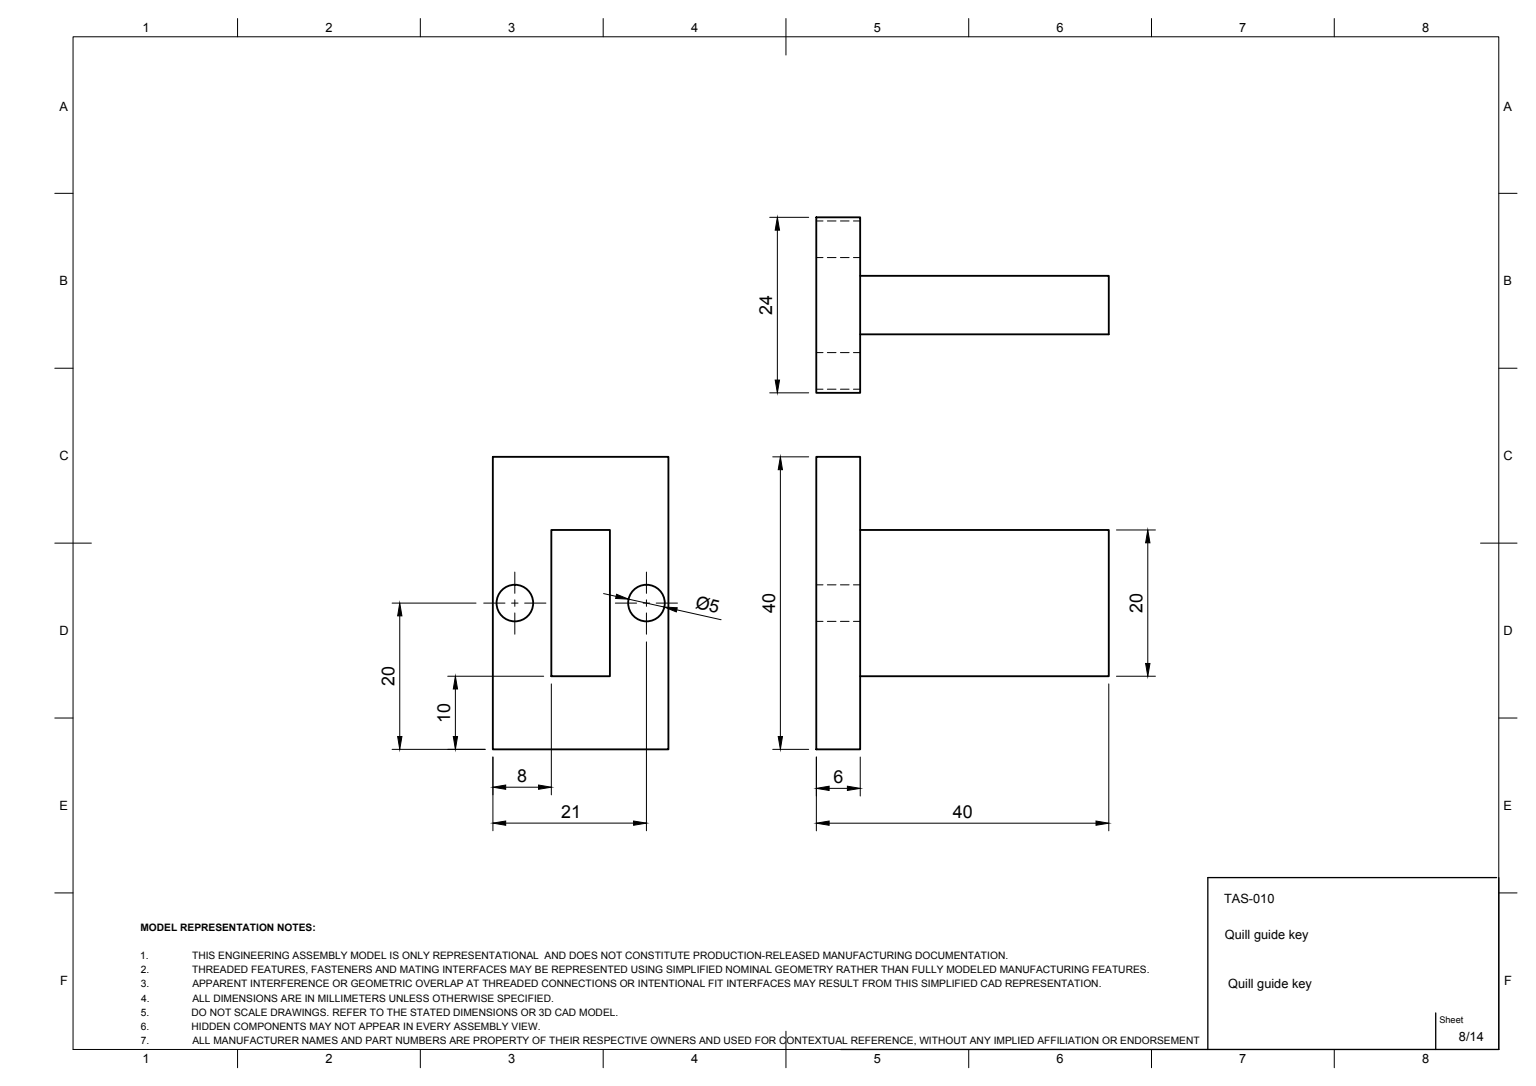
ISO-10303-21;
HEADER;
/* Generated by software containing ST-Developer
 * from STEP Tools, Inc. (www.steptools.com) 
 */

FILE_DESCRIPTION(
/* description */ (
'Independent keyed-quill tailstock, native coupled50mm slider andM16x2
 feed screw, conical dead center, bronze sleeves/thrust washers, cross
-pinned handwheel and bolted guide key. Custom center taper; no standa
rd taper compatibility, machine-bed compatibility or load rating assig
ned.'),
/* implementation_level */ '2;1');

FILE_NAME(
/* name */ 'Quill guide key.step',
/* time_stamp */ '2026-11-14T07:17:36-08:00',
/* author */ (''),
/* organization */ (''),
/* preprocessor_version */ 'ST-DEVELOPER v20.2',
/* originating_system */ 'Autodesk Translation Framework v15.17.0.0',
/* authorisation */ '');

FILE_SCHEMA (('AUTOMOTIVE_DESIGN { 1 0 10303 214 3 1 1 }'));
ENDSEC;

DATA;
#10=MECHANICAL_DESIGN_GEOMETRIC_PRESENTATION_REPRESENTATION('',(#158),#289387);
#124=SHAPE_REPRESENTATION_RELATIONSHIP('SRR','None',#289459,#141);
#141=ADVANCED_BREP_SHAPE_REPRESENTATION('',(#175),#289375);
#158=STYLED_ITEM('',(#289552),#175);
#175=MANIFOLD_SOLID_BREP('Body1',#16846);
#223=FACE_BOUND('',#1527,.T.);
#224=FACE_BOUND('',#1528,.T.);
#225=FACE_BOUND('',#1529,.T.);
#226=FACE_BOUND('',#1535,.T.);
#227=FACE_BOUND('',#1536,.T.);
#354=PLANE('',#17542);
#355=PLANE('',#17543);
#356=PLANE('',#17544);
#357=PLANE('',#17545);
#358=PLANE('',#17546);
#359=PLANE('',#17547);
#360=PLANE('',#17548);
#361=PLANE('',#17549);
#362=PLANE('',#17550);
#363=PLANE('',#17551);
#364=PLANE('',#17552);
#838=FACE_OUTER_BOUND('',#1524,.T.);
#839=FACE_OUTER_BOUND('',#1525,.T.);
#840=FACE_OUTER_BOUND('',#1526,.T.);
#841=FACE_OUTER_BOUND('',#1530,.T.);
#842=FACE_OUTER_BOUND('',#1531,.T.);
#843=FACE_OUTER_BOUND('',#1532,.T.);
#844=FACE_OUTER_BOUND('',#1533,.T.);
#845=FACE_OUTER_BOUND('',#1534,.T.);
#846=FACE_OUTER_BOUND('',#1537,.T.);
#847=FACE_OUTER_BOUND('',#1538,.T.);
#848=FACE_OUTER_BOUND('',#1539,.T.);
#849=FACE_OUTER_BOUND('',#1540,.T.);
#850=FACE_OUTER_BOUND('',#1541,.T.);
#1524=EDGE_LOOP('',(#13673,#13674,#13675,#13676));
#1525=EDGE_LOOP('',(#13677,#13678,#13679,#13680));
#1526=EDGE_LOOP('',(#13681,#13682,#13683,#13684));
#1527=EDGE_LOOP('',(#13685));
#1528=EDGE_LOOP('',(#13686));
#1529=EDGE_LOOP('',(#13687,#13688,#13689,#13690));
#1530=EDGE_LOOP('',(#13691,#13692,#13693,#13694));
#1531=EDGE_LOOP('',(#13695,#13696,#13697,#13698));
#1532=EDGE_LOOP('',(#13699,#13700,#13701,#13702));
#1533=EDGE_LOOP('',(#13703,#13704,#13705,#13706));
#1534=EDGE_LOOP('',(#13707,#13708,#13709,#13710));
#1535=EDGE_LOOP('',(#13711));
#1536=EDGE_LOOP('',(#13712));
#1537=EDGE_LOOP('',(#13713,#13714,#13715,#13716));
#1538=EDGE_LOOP('',(#13717,#13718,#13719,#13720));
#1539=EDGE_LOOP('',(#13721,#13722,#13723,#13724));
#1540=EDGE_LOOP('',(#13725,#13726,#13727,#13728));
#1541=EDGE_LOOP('',(#13729,#13730,#13731,#13732));
#1899=CIRCLE('',#17537,2.5);
#1900=CIRCLE('',#17538,2.5);
#1901=CIRCLE('',#17540,2.5);
#1902=CIRCLE('',#17541,2.5);
#4329=LINE('',#185169,#4966);
#4330=LINE('',#185175,#4967);
#4331=LINE('',#185180,#4968);
#4332=LINE('',#185182,#4969);
#4333=LINE('',#185184,#4970);
#4334=LINE('',#185185,#4971);
#4335=LINE('',#185188,#4972);
#4336=LINE('',#185190,#4973);
#4337=LINE('',#185192,#4974);
#4338=LINE('',#185193,#4975);
#4339=LINE('',#185196,#4976);
#4340=LINE('',#185198,#4977);
#4341=LINE('',#185199,#4978);
#4342=LINE('',#185202,#4979);
#4343=LINE('',#185203,#4980);
#4344=LINE('',#185206,#4981);
#4345=LINE('',#185207,#4982);
#4346=LINE('',#185209,#4983);
#4347=LINE('',#185214,#4984);
#4348=LINE('',#185215,#4985);
#4349=LINE('',#185216,#4986);
#4350=LINE('',#185219,#4987);
#4351=LINE('',#185220,#4988);
#4352=LINE('',#185223,#4989);
#4353=LINE('',#185224,#4990);
#4354=LINE('',#185226,#4991);
#4966=VECTOR('',#19261,2.5);
#4967=VECTOR('',#19268,2.5);
#4968=VECTOR('',#19273,10.);
#4969=VECTOR('',#19274,10.);
#4970=VECTOR('',#19275,10.);
#4971=VECTOR('',#19276,10.);
#4972=VECTOR('',#19277,10.);
#4973=VECTOR('',#19278,10.);
#4974=VECTOR('',#19279,10.);
#4975=VECTOR('',#19280,10.);
#4976=VECTOR('',#19283,10.);
#4977=VECTOR('',#19284,10.);
#4978=VECTOR('',#19285,10.);
#4979=VECTOR('',#19288,10.);
#4980=VECTOR('',#19289,10.);
#4981=VECTOR('',#19292,10.);
#4982=VECTOR('',#19293,10.);
#4983=VECTOR('',#19296,10.);
#4984=VECTOR('',#19301,10.);
#4985=VECTOR('',#19302,10.);
#4986=VECTOR('',#19303,10.);
#4987=VECTOR('',#19306,10.);
#4988=VECTOR('',#19307,10.);
#4989=VECTOR('',#19310,10.);
#4990=VECTOR('',#19311,10.);
#4991=VECTOR('',#19314,10.);
#6580=VERTEX_POINT('',#185166);
#6581=VERTEX_POINT('',#185168);
#6582=VERTEX_POINT('',#185172);
#6583=VERTEX_POINT('',#185174);
#6584=VERTEX_POINT('',#185178);
#6585=VERTEX_POINT('',#185179);
#6586=VERTEX_POINT('',#185181);
#6587=VERTEX_POINT('',#185183);
#6588=VERTEX_POINT('',#185186);
#6589=VERTEX_POINT('',#185187);
#6590=VERTEX_POINT('',#185189);
#6591=VERTEX_POINT('',#185191);
#6592=VERTEX_POINT('',#185195);
#6593=VERTEX_POINT('',#185197);
#6594=VERTEX_POINT('',#185201);
#6595=VERTEX_POINT('',#185205);
#6596=VERTEX_POINT('',#185212);
#6597=VERTEX_POINT('',#185213);
#6598=VERTEX_POINT('',#185218);
#6599=VERTEX_POINT('',#185222);
#9148=EDGE_CURVE('',#6580,#6580,#1899,.T.);
#9149=EDGE_CURVE('',#6580,#6581,#4329,.T.);
#9150=EDGE_CURVE('',#6581,#6581,#1900,.T.);
#9151=EDGE_CURVE('',#6582,#6582,#1901,.T.);
#9152=EDGE_CURVE('',#6582,#6583,#4330,.T.);
#9153=EDGE_CURVE('',#6583,#6583,#1902,.T.);
#9154=EDGE_CURVE('',#6584,#6585,#4331,.T.);
#9155=EDGE_CURVE('',#6586,#6584,#4332,.T.);
#9156=EDGE_CURVE('',#6587,#6586,#4333,.T.);
#9157=EDGE_CURVE('',#6585,#6587,#4334,.T.);
#9158=EDGE_CURVE('',#6588,#6589,#4335,.T.);
#9159=EDGE_CURVE('',#6589,#6590,#4336,.T.);
#9160=EDGE_CURVE('',#6590,#6591,#4337,.T.);
#9161=EDGE_CURVE('',#6591,#6588,#4338,.T.);
#9162=EDGE_CURVE('',#6584,#6592,#4339,.T.);
#9163=EDGE_CURVE('',#6593,#6592,#4340,.T.);
#9164=EDGE_CURVE('',#6586,#6593,#4341,.T.);
#9165=EDGE_CURVE('',#6594,#6593,#4342,.T.);
#9166=EDGE_CURVE('',#6587,#6594,#4343,.T.);
#9167=EDGE_CURVE('',#6595,#6594,#4344,.T.);
#9168=EDGE_CURVE('',#6585,#6595,#4345,.T.);
#9169=EDGE_CURVE('',#6592,#6595,#4346,.T.);
#9170=EDGE_CURVE('',#6596,#6597,#4347,.T.);
#9171=EDGE_CURVE('',#6597,#6589,#4348,.T.);
#9172=EDGE_CURVE('',#6596,#6588,#4349,.T.);
#9173=EDGE_CURVE('',#6598,#6596,#4350,.T.);
#9174=EDGE_CURVE('',#6598,#6591,#4351,.T.);
#9175=EDGE_CURVE('',#6599,#6598,#4352,.T.);
#9176=EDGE_CURVE('',#6599,#6590,#4353,.T.);
#9177=EDGE_CURVE('',#6597,#6599,#4354,.T.);
#13673=ORIENTED_EDGE('',*,*,#9148,.F.);
#13674=ORIENTED_EDGE('',*,*,#9149,.T.);
#13675=ORIENTED_EDGE('',*,*,#9150,.F.);
#13676=ORIENTED_EDGE('',*,*,#9149,.F.);
#13677=ORIENTED_EDGE('',*,*,#9151,.F.);
#13678=ORIENTED_EDGE('',*,*,#9152,.T.);
#13679=ORIENTED_EDGE('',*,*,#9153,.F.);
#13680=ORIENTED_EDGE('',*,*,#9152,.F.);
#13681=ORIENTED_EDGE('',*,*,#9154,.F.);
#13682=ORIENTED_EDGE('',*,*,#9155,.F.);
#13683=ORIENTED_EDGE('',*,*,#9156,.F.);
#13684=ORIENTED_EDGE('',*,*,#9157,.F.);
#13685=ORIENTED_EDGE('',*,*,#9150,.T.);
#13686=ORIENTED_EDGE('',*,*,#9153,.T.);
#13687=ORIENTED_EDGE('',*,*,#9158,.T.);
#13688=ORIENTED_EDGE('',*,*,#9159,.T.);
#13689=ORIENTED_EDGE('',*,*,#9160,.T.);
#13690=ORIENTED_EDGE('',*,*,#9161,.T.);
#13691=ORIENTED_EDGE('',*,*,#9155,.T.);
#13692=ORIENTED_EDGE('',*,*,#9162,.T.);
#13693=ORIENTED_EDGE('',*,*,#9163,.F.);
#13694=ORIENTED_EDGE('',*,*,#9164,.F.);
#13695=ORIENTED_EDGE('',*,*,#9156,.T.);
#13696=ORIENTED_EDGE('',*,*,#9164,.T.);
#13697=ORIENTED_EDGE('',*,*,#9165,.F.);
#13698=ORIENTED_EDGE('',*,*,#9166,.F.);
#13699=ORIENTED_EDGE('',*,*,#9157,.T.);
#13700=ORIENTED_EDGE('',*,*,#9166,.T.);
#13701=ORIENTED_EDGE('',*,*,#9167,.F.);
#13702=ORIENTED_EDGE('',*,*,#9168,.F.);
#13703=ORIENTED_EDGE('',*,*,#9154,.T.);
#13704=ORIENTED_EDGE('',*,*,#9168,.T.);
#13705=ORIENTED_EDGE('',*,*,#9169,.F.);
#13706=ORIENTED_EDGE('',*,*,#9162,.F.);
#13707=ORIENTED_EDGE('',*,*,#9169,.T.);
#13708=ORIENTED_EDGE('',*,*,#9167,.T.);
#13709=ORIENTED_EDGE('',*,*,#9165,.T.);
#13710=ORIENTED_EDGE('',*,*,#9163,.T.);
#13711=ORIENTED_EDGE('',*,*,#9148,.T.);
#13712=ORIENTED_EDGE('',*,*,#9151,.T.);
#13713=ORIENTED_EDGE('',*,*,#9170,.T.);
#13714=ORIENTED_EDGE('',*,*,#9171,.T.);
#13715=ORIENTED_EDGE('',*,*,#9158,.F.);
#13716=ORIENTED_EDGE('',*,*,#9172,.F.);
#13717=ORIENTED_EDGE('',*,*,#9173,.T.);
#13718=ORIENTED_EDGE('',*,*,#9172,.T.);
#13719=ORIENTED_EDGE('',*,*,#9161,.F.);
#13720=ORIENTED_EDGE('',*,*,#9174,.F.);
#13721=ORIENTED_EDGE('',*,*,#9175,.T.);
#13722=ORIENTED_EDGE('',*,*,#9174,.T.);
#13723=ORIENTED_EDGE('',*,*,#9160,.F.);
#13724=ORIENTED_EDGE('',*,*,#9176,.F.);
#13725=ORIENTED_EDGE('',*,*,#9177,.T.);
#13726=ORIENTED_EDGE('',*,*,#9176,.T.);
#13727=ORIENTED_EDGE('',*,*,#9159,.F.);
#13728=ORIENTED_EDGE('',*,*,#9171,.F.);
#13729=ORIENTED_EDGE('',*,*,#9177,.F.);
#13730=ORIENTED_EDGE('',*,*,#9170,.F.);
#13731=ORIENTED_EDGE('',*,*,#9173,.F.);
#13732=ORIENTED_EDGE('',*,*,#9175,.F.);
#16038=CYLINDRICAL_SURFACE('',#17536,2.5);
#16039=CYLINDRICAL_SURFACE('',#17539,2.5);
#16606=ADVANCED_FACE('',(#838),#16038,.F.);
#16607=ADVANCED_FACE('',(#839),#16039,.F.);
#16608=ADVANCED_FACE('',(#840,#223,#224,#225),#354,.F.);
#16609=ADVANCED_FACE('',(#841),#355,.T.);
#16610=ADVANCED_FACE('',(#842),#356,.T.);
#16611=ADVANCED_FACE('',(#843),#357,.T.);
#16612=ADVANCED_FACE('',(#844),#358,.T.);
#16613=ADVANCED_FACE('',(#845,#226,#227),#359,.T.);
#16614=ADVANCED_FACE('',(#846),#360,.T.);
#16615=ADVANCED_FACE('',(#847),#361,.T.);
#16616=ADVANCED_FACE('',(#848),#362,.T.);
#16617=ADVANCED_FACE('',(#849),#363,.T.);
#16618=ADVANCED_FACE('',(#850),#364,.F.);
#16846=CLOSED_SHELL('',(#16606,#16607,#16608,#16609,#16610,#16611,#16612,
#16613,#16614,#16615,#16616,#16617,#16618));
#17535=AXIS2_PLACEMENT_3D('',#185164,#19255,#19256);
#17536=AXIS2_PLACEMENT_3D('',#185165,#19257,#19258);
#17537=AXIS2_PLACEMENT_3D('',#185167,#19259,#19260);
#17538=AXIS2_PLACEMENT_3D('',#185170,#19262,#19263);
#17539=AXIS2_PLACEMENT_3D('',#185171,#19264,#19265);
#17540=AXIS2_PLACEMENT_3D('',#185173,#19266,#19267);
#17541=AXIS2_PLACEMENT_3D('',#185176,#19269,#19270);
#17542=AXIS2_PLACEMENT_3D('',#185177,#19271,#19272);
#17543=AXIS2_PLACEMENT_3D('',#185194,#19281,#19282);
#17544=AXIS2_PLACEMENT_3D('',#185200,#19286,#19287);
#17545=AXIS2_PLACEMENT_3D('',#185204,#19290,#19291);
#17546=AXIS2_PLACEMENT_3D('',#185208,#19294,#19295);
#17547=AXIS2_PLACEMENT_3D('',#185210,#19297,#19298);
#17548=AXIS2_PLACEMENT_3D('',#185211,#19299,#19300);
#17549=AXIS2_PLACEMENT_3D('',#185217,#19304,#19305);
#17550=AXIS2_PLACEMENT_3D('',#185221,#19308,#19309);
#17551=AXIS2_PLACEMENT_3D('',#185225,#19312,#19313);
#17552=AXIS2_PLACEMENT_3D('',#185227,#19315,#19316);
#19255=DIRECTION('axis',(0.,0.,1.));
#19256=DIRECTION('refdir',(1.,0.,0.));
#19257=DIRECTION('center_axis',(0.,0.,-1.));
#19258=DIRECTION('ref_axis',(1.,0.,0.));
#19259=DIRECTION('center_axis',(0.,0.,-1.));
#19260=DIRECTION('ref_axis',(1.,0.,0.));
#19261=DIRECTION('',(0.,0.,-1.));
#19262=DIRECTION('center_axis',(0.,0.,1.));
#19263=DIRECTION('ref_axis',(1.,0.,0.));
#19264=DIRECTION('center_axis',(0.,0.,-1.));
#19265=DIRECTION('ref_axis',(1.,0.,0.));
#19266=DIRECTION('center_axis',(0.,0.,-1.));
#19267=DIRECTION('ref_axis',(1.,0.,0.));
#19268=DIRECTION('',(0.,0.,-1.));
#19269=DIRECTION('center_axis',(0.,0.,1.));
#19270=DIRECTION('ref_axis',(1.,0.,0.));
#19271=DIRECTION('center_axis',(0.,0.,1.));
#19272=DIRECTION('ref_axis',(1.,0.,0.));
#19273=DIRECTION('',(0.,-1.,0.));
#19274=DIRECTION('',(-1.,0.,0.));
#19275=DIRECTION('',(0.,1.,0.));
#19276=DIRECTION('',(1.,0.,0.));
#19277=DIRECTION('',(-1.,0.,0.));
#19278=DIRECTION('',(0.,-1.,0.));
#19279=DIRECTION('',(1.,0.,0.));
#19280=DIRECTION('',(0.,1.,0.));
#19281=DIRECTION('center_axis',(0.,1.,0.));
#19282=DIRECTION('ref_axis',(-1.,0.,0.));
#19283=DIRECTION('',(0.,0.,1.));
#19284=DIRECTION('',(-1.,0.,0.));
#19285=DIRECTION('',(0.,0.,1.));
#19286=DIRECTION('center_axis',(1.,0.,0.));
#19287=DIRECTION('ref_axis',(0.,1.,0.));
#19288=DIRECTION('',(0.,1.,0.));
#19289=DIRECTION('',(0.,0.,1.));
#19290=DIRECTION('center_axis',(0.,-1.,0.));
#19291=DIRECTION('ref_axis',(1.,0.,0.));
#19292=DIRECTION('',(1.,0.,0.));
#19293=DIRECTION('',(0.,0.,1.));
#19294=DIRECTION('center_axis',(-1.,0.,0.));
#19295=DIRECTION('ref_axis',(0.,-1.,0.));
#19296=DIRECTION('',(0.,-1.,0.));
#19297=DIRECTION('center_axis',(0.,0.,1.));
#19298=DIRECTION('ref_axis',(1.,0.,0.));
#19299=DIRECTION('center_axis',(0.,1.,0.));
#19300=DIRECTION('ref_axis',(-1.,0.,0.));
#19301=DIRECTION('',(-1.,0.,0.));
#19302=DIRECTION('',(0.,0.,1.));
#19303=DIRECTION('',(0.,0.,1.));
#19304=DIRECTION('center_axis',(1.,0.,0.));
#19305=DIRECTION('ref_axis',(0.,1.,0.));
#19306=DIRECTION('',(0.,1.,0.));
#19307=DIRECTION('',(0.,0.,1.));
#19308=DIRECTION('center_axis',(0.,-1.,0.));
#19309=DIRECTION('ref_axis',(1.,0.,0.));
#19310=DIRECTION('',(1.,0.,0.));
#19311=DIRECTION('',(0.,0.,1.));
#19312=DIRECTION('center_axis',(-1.,0.,0.));
#19313=DIRECTION('ref_axis',(0.,-1.,0.));
#19314=DIRECTION('',(0.,-1.,0.));
#19315=DIRECTION('center_axis',(0.,0.,1.));
#19316=DIRECTION('ref_axis',(1.,0.,0.));
#185164=CARTESIAN_POINT('',(0.,0.,0.));
#185165=CARTESIAN_POINT('Origin',(80.,-9.,143.));
#185166=CARTESIAN_POINT('',(77.5,-9.,146.));
#185167=CARTESIAN_POINT('Origin',(80.,-9.,146.));
#185168=CARTESIAN_POINT('',(77.5,-9.,140.));
#185169=CARTESIAN_POINT('',(77.5,-9.,143.));
#185170=CARTESIAN_POINT('Origin',(80.,-9.,140.));
#185171=CARTESIAN_POINT('Origin',(80.,9.,143.));
#185172=CARTESIAN_POINT('',(77.5,9.,146.));
#185173=CARTESIAN_POINT('Origin',(80.,9.,146.));
#185174=CARTESIAN_POINT('',(77.5,9.,140.));
#185175=CARTESIAN_POINT('',(77.5,9.,143.));
#185176=CARTESIAN_POINT('Origin',(80.,9.,140.));
#185177=CARTESIAN_POINT('Origin',(80.,0.,140.));
#185178=CARTESIAN_POINT('',(60.,12.,140.));
#185179=CARTESIAN_POINT('',(60.,-12.,140.));
#185180=CARTESIAN_POINT('',(60.,12.,140.));
#185181=CARTESIAN_POINT('',(100.,12.,140.));
#185182=CARTESIAN_POINT('',(100.,12.,140.));
#185183=CARTESIAN_POINT('',(100.,-12.,140.));
#185184=CARTESIAN_POINT('',(100.,-12.,140.));
#185185=CARTESIAN_POINT('',(60.,-12.,140.));
#185186=CARTESIAN_POINT('',(90.,4.,140.));
#185187=CARTESIAN_POINT('',(70.,4.,140.));
#185188=CARTESIAN_POINT('',(90.,4.,140.));
#185189=CARTESIAN_POINT('',(70.,-4.,140.));
#185190=CARTESIAN_POINT('',(70.,4.,140.));
#185191=CARTESIAN_POINT('',(90.,-4.,140.));
#185192=CARTESIAN_POINT('',(70.,-4.,140.));
#185193=CARTESIAN_POINT('',(90.,-4.,140.));
#185194=CARTESIAN_POINT('Origin',(100.,12.,140.));
#185195=CARTESIAN_POINT('',(60.,12.,146.));
#185196=CARTESIAN_POINT('',(60.,12.,140.));
#185197=CARTESIAN_POINT('',(100.,12.,146.));
#185198=CARTESIAN_POINT('',(100.,12.,146.));
#185199=CARTESIAN_POINT('',(100.,12.,140.));
#185200=CARTESIAN_POINT('Origin',(100.,-12.,140.));
#185201=CARTESIAN_POINT('',(100.,-12.,146.));
#185202=CARTESIAN_POINT('',(100.,-12.,146.));
#185203=CARTESIAN_POINT('',(100.,-12.,140.));
#185204=CARTESIAN_POINT('Origin',(60.,-12.,140.));
#185205=CARTESIAN_POINT('',(60.,-12.,146.));
#185206=CARTESIAN_POINT('',(60.,-12.,146.));
#185207=CARTESIAN_POINT('',(60.,-12.,140.));
#185208=CARTESIAN_POINT('Origin',(60.,12.,140.));
#185209=CARTESIAN_POINT('',(60.,12.,146.));
#185210=CARTESIAN_POINT('Origin',(80.,0.,146.));
#185211=CARTESIAN_POINT('Origin',(90.,4.,106.));
#185212=CARTESIAN_POINT('',(90.,4.,106.));
#185213=CARTESIAN_POINT('',(70.,4.,106.));
#185214=CARTESIAN_POINT('',(90.,4.,106.));
#185215=CARTESIAN_POINT('',(70.,4.,106.));
#185216=CARTESIAN_POINT('',(90.,4.,106.));
#185217=CARTESIAN_POINT('Origin',(90.,-4.,106.));
#185218=CARTESIAN_POINT('',(90.,-4.,106.));
#185219=CARTESIAN_POINT('',(90.,-4.,106.));
#185220=CARTESIAN_POINT('',(90.,-4.,106.));
#185221=CARTESIAN_POINT('Origin',(70.,-4.,106.));
#185222=CARTESIAN_POINT('',(70.,-4.,106.));
#185223=CARTESIAN_POINT('',(70.,-4.,106.));
#185224=CARTESIAN_POINT('',(70.,-4.,106.));
#185225=CARTESIAN_POINT('Origin',(70.,4.,106.));
#185226=CARTESIAN_POINT('',(70.,4.,106.));
#185227=CARTESIAN_POINT('Origin',(80.,0.,106.));
#289356=UNCERTAINTY_MEASURE_WITH_UNIT(LENGTH_MEASURE(0.01),#289388,
'DISTANCE_ACCURACY_VALUE',
'Maximum model space distance between geometric entities at asserted c
onnectivities');
#289368=UNCERTAINTY_MEASURE_WITH_UNIT(LENGTH_MEASURE(0.01),#289388,
'DISTANCE_ACCURACY_VALUE',
'Maximum model space distance between geometric entities at asserted c
onnectivities');
#289375=(
GEOMETRIC_REPRESENTATION_CONTEXT(3)
GLOBAL_UNCERTAINTY_ASSIGNED_CONTEXT((#289356))
GLOBAL_UNIT_ASSIGNED_CONTEXT((#289388,#289390,#289391))
REPRESENTATION_CONTEXT('','3D')
);
#289387=(
GEOMETRIC_REPRESENTATION_CONTEXT(3)
GLOBAL_UNCERTAINTY_ASSIGNED_CONTEXT((#289368))
GLOBAL_UNIT_ASSIGNED_CONTEXT((#289388,#289390,#289391))
REPRESENTATION_CONTEXT('','3D')
);
#289388=(
LENGTH_UNIT()
NAMED_UNIT(*)
SI_UNIT(.MILLI.,.METRE.)
);
#289390=(
NAMED_UNIT(*)
PLANE_ANGLE_UNIT()
SI_UNIT($,.RADIAN.)
);
#289391=(
NAMED_UNIT(*)
SI_UNIT($,.STERADIAN.)
SOLID_ANGLE_UNIT()
);
#289398=SHAPE_DEFINITION_REPRESENTATION(#289416,#289459);
#289416=PRODUCT_DEFINITION_SHAPE('',$,#289478);
#289459=SHAPE_REPRESENTATION('',(#17535),#289375);
#289471=PRODUCT_DEFINITION_CONTEXT('part definition',#289527,'design');
#289478=PRODUCT_DEFINITION('Quill guide key','Quill guide key',#289496,
#289471);
#289496=PRODUCT_DEFINITION_FORMATION('',$,#289535);
#289527=APPLICATION_CONTEXT(
'Core Data for Automotive Mechanical Design Process');
#289528=PRODUCT_CONTEXT('part definition',#289527,'mechanical');
#289535=PRODUCT('Quill guide key','Quill guide key',$,(#289528));
#289552=PRESENTATION_STYLE_ASSIGNMENT((#289559));
#289559=SURFACE_STYLE_USAGE(.BOTH.,#289566);
#289566=SURFACE_SIDE_STYLE('',(#289573));
#289573=SURFACE_STYLE_FILL_AREA(#289580);
#289580=FILL_AREA_STYLE('Opaque(81,175,227)',(#289587));
#289587=FILL_AREA_STYLE_COLOUR('Opaque(81,175,227)',#289594);
#289594=COLOUR_RGB('Opaque(81,175,227)',0.317647058823529,0.686274509803922,
0.890196078431372);
ENDSEC;
END-ISO-10303-21;
